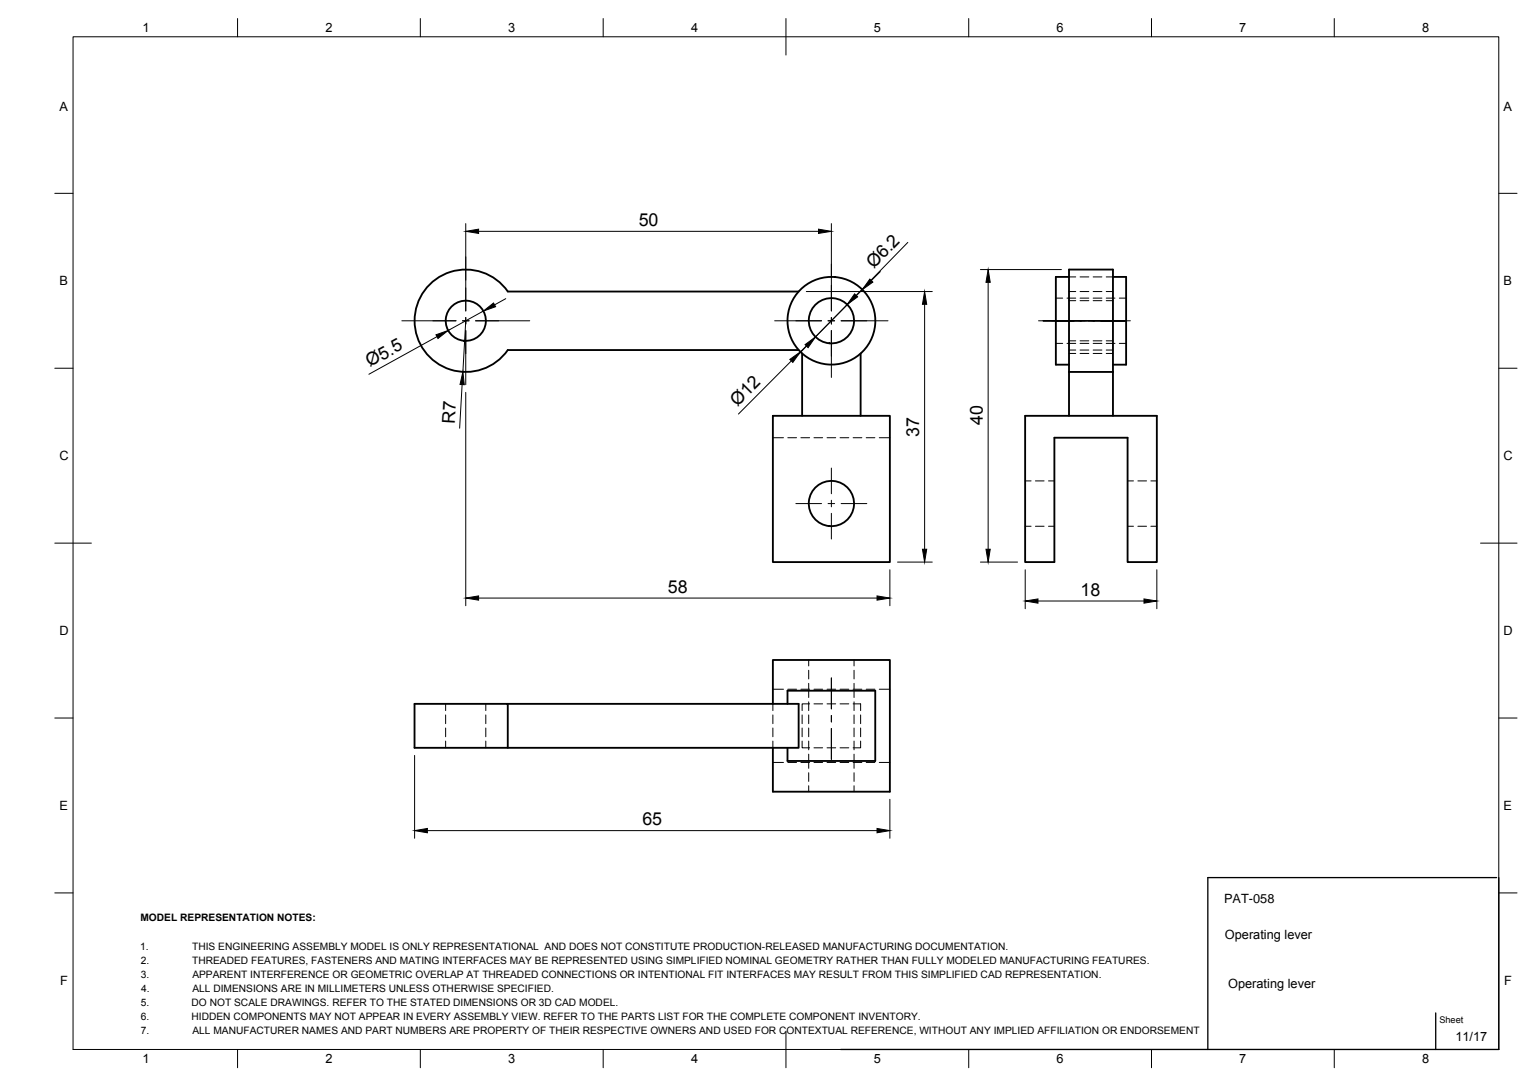
ISO-10303-21;
HEADER;
/* Generated by software containing ST-Developer
 * from STEP Tools, Inc. (www.steptools.com) 
 */

FILE_DESCRIPTION(
/* description */ ('Horizontal push-pull toggle clamp'),
/* implementation_level */ '2;1');

FILE_NAME(
/* name */ 'Operating lever.step',
/* time_stamp */ '2026-10-27T21:21:09-07:00',
/* author */ (''),
/* organization */ (''),
/* preprocessor_version */ 'ST-DEVELOPER v20.2',
/* originating_system */ 'Autodesk Translation Framework v15.17.0.0',
/* authorisation */ '');

FILE_SCHEMA (('AUTOMOTIVE_DESIGN { 1 0 10303 214 3 1 1 }'));
ENDSEC;

DATA;
#10=MECHANICAL_DESIGN_GEOMETRIC_PRESENTATION_REPRESENTATION('',(#186),#4791);
#160=SHAPE_REPRESENTATION_RELATIONSHIP('SRR','None',#4864,#173);
#173=ADVANCED_BREP_SHAPE_REPRESENTATION('',(#199),#4777);
#186=STYLED_ITEM('',(#5009),#199);
#199=MANIFOLD_SOLID_BREP('Body1',#2630);
#223=FACE_BOUND('',#563,.T.);
#224=FACE_BOUND('',#566,.T.);
#225=FACE_BOUND('',#572,.T.);
#226=FACE_BOUND('',#575,.T.);
#227=FACE_BOUND('',#581,.T.);
#228=FACE_BOUND('',#582,.T.);
#229=FACE_BOUND('',#584,.T.);
#230=FACE_BOUND('',#586,.T.);
#231=FACE_BOUND('',#589,.T.);
#232=FACE_BOUND('',#591,.T.);
#233=FACE_BOUND('',#595,.T.);
#283=PLANE('',#2848);
#284=PLANE('',#2850);
#285=PLANE('',#2851);
#286=PLANE('',#2853);
#287=PLANE('',#2860);
#288=PLANE('',#2861);
#289=PLANE('',#2862);
#290=PLANE('',#2863);
#291=PLANE('',#2864);
#292=PLANE('',#2866);
#293=PLANE('',#2867);
#294=PLANE('',#2869);
#295=PLANE('',#2873);
#296=PLANE('',#2874);
#297=PLANE('',#2875);
#298=PLANE('',#2876);
#299=PLANE('',#2877);
#300=PLANE('',#2878);
#301=PLANE('',#2879);
#302=PLANE('',#2880);
#395=FACE_OUTER_BOUND('',#559,.T.);
#396=FACE_OUTER_BOUND('',#560,.T.);
#397=FACE_OUTER_BOUND('',#561,.T.);
#398=FACE_OUTER_BOUND('',#562,.T.);
#399=FACE_OUTER_BOUND('',#564,.T.);
#400=FACE_OUTER_BOUND('',#565,.T.);
#401=FACE_OUTER_BOUND('',#567,.T.);
#402=FACE_OUTER_BOUND('',#568,.T.);
#403=FACE_OUTER_BOUND('',#569,.T.);
#404=FACE_OUTER_BOUND('',#570,.T.);
#405=FACE_OUTER_BOUND('',#571,.T.);
#406=FACE_OUTER_BOUND('',#573,.T.);
#407=FACE_OUTER_BOUND('',#574,.T.);
#408=FACE_OUTER_BOUND('',#576,.T.);
#409=FACE_OUTER_BOUND('',#577,.T.);
#410=FACE_OUTER_BOUND('',#578,.T.);
#411=FACE_OUTER_BOUND('',#579,.T.);
#412=FACE_OUTER_BOUND('',#580,.T.);
#413=FACE_OUTER_BOUND('',#583,.T.);
#414=FACE_OUTER_BOUND('',#585,.T.);
#415=FACE_OUTER_BOUND('',#587,.T.);
#416=FACE_OUTER_BOUND('',#588,.T.);
#417=FACE_OUTER_BOUND('',#590,.T.);
#418=FACE_OUTER_BOUND('',#592,.T.);
#419=FACE_OUTER_BOUND('',#593,.T.);
#420=FACE_OUTER_BOUND('',#594,.T.);
#559=EDGE_LOOP('',(#1951,#1952,#1953,#1954));
#560=EDGE_LOOP('',(#1955,#1956,#1957,#1958));
#561=EDGE_LOOP('',(#1959,#1960,#1961,#1962));
#562=EDGE_LOOP('',(#1963,#1964,#1965,#1966));
#563=EDGE_LOOP('',(#1967));
#564=EDGE_LOOP('',(#1968,#1969,#1970,#1971));
#565=EDGE_LOOP('',(#1972,#1973,#1974,#1975));
#566=EDGE_LOOP('',(#1976));
#567=EDGE_LOOP('',(#1977,#1978,#1979,#1980));
#568=EDGE_LOOP('',(#1981,#1982,#1983,#1984));
#569=EDGE_LOOP('',(#1985,#1986,#1987,#1988));
#570=EDGE_LOOP('',(#1989,#1990,#1991,#1992));
#571=EDGE_LOOP('',(#1993,#1994,#1995,#1996));
#572=EDGE_LOOP('',(#1997));
#573=EDGE_LOOP('',(#1998,#1999,#2000,#2001));
#574=EDGE_LOOP('',(#2002,#2003,#2004,#2005));
#575=EDGE_LOOP('',(#2006));
#576=EDGE_LOOP('',(#2007,#2008,#2009,#2010));
#577=EDGE_LOOP('',(#2011,#2012,#2013,#2014));
#578=EDGE_LOOP('',(#2015,#2016,#2017,#2018));
#579=EDGE_LOOP('',(#2019,#2020,#2021,#2022));
#580=EDGE_LOOP('',(#2023,#2024,#2025,#2026));
#581=EDGE_LOOP('',(#2027,#2028,#2029,#2030));
#582=EDGE_LOOP('',(#2031,#2032,#2033,#2034));
#583=EDGE_LOOP('',(#2035));
#584=EDGE_LOOP('',(#2036));
#585=EDGE_LOOP('',(#2037));
#586=EDGE_LOOP('',(#2038));
#587=EDGE_LOOP('',(#2039,#2040,#2041,#2042,#2043,#2044,#2045,#2046));
#588=EDGE_LOOP('',(#2047,#2048,#2049,#2050));
#589=EDGE_LOOP('',(#2051));
#590=EDGE_LOOP('',(#2052,#2053,#2054,#2055));
#591=EDGE_LOOP('',(#2056,#2057,#2058,#2059));
#592=EDGE_LOOP('',(#2060,#2061,#2062,#2063));
#593=EDGE_LOOP('',(#2064,#2065,#2066,#2067,#2068,#2069,#2070,#2071));
#594=EDGE_LOOP('',(#2072,#2073,#2074,#2075));
#595=EDGE_LOOP('',(#2076));
#724=CIRCLE('',#2840,0.275);
#725=CIRCLE('',#2841,0.275);
#726=CIRCLE('',#2843,0.31);
#727=CIRCLE('',#2844,0.31);
#728=CIRCLE('',#2846,0.7);
#729=CIRCLE('',#2847,0.7);
#730=CIRCLE('',#2849,0.6);
#731=CIRCLE('',#2852,0.6);
#732=CIRCLE('',#2855,0.31);
#733=CIRCLE('',#2856,0.31);
#734=CIRCLE('',#2858,0.31);
#735=CIRCLE('',#2859,0.31);
#736=CIRCLE('',#2865,0.6);
#737=CIRCLE('',#2868,0.6);
#738=CIRCLE('',#2871,0.6);
#739=CIRCLE('',#2872,0.6);
#866=LINE('',#4038,#1086);
#867=LINE('',#4044,#1087);
#868=LINE('',#4049,#1088);
#869=LINE('',#4053,#1089);
#870=LINE('',#4057,#1090);
#871=LINE('',#4060,#1091);
#872=LINE('',#4063,#1092);
#873=LINE('',#4064,#1093);
#874=LINE('',#4067,#1094);
#875=LINE('',#4070,#1095);
#876=LINE('',#4075,#1096);
#877=LINE('',#4081,#1097);
#878=LINE('',#4086,#1098);
#879=LINE('',#4088,#1099);
#880=LINE('',#4090,#1100);
#881=LINE('',#4091,#1101);
#882=LINE('',#4095,#1102);
#883=LINE('',#4097,#1103);
#884=LINE('',#4099,#1104);
#885=LINE('',#4100,#1105);
#886=LINE('',#4104,#1106);
#887=LINE('',#4105,#1107);
#888=LINE('',#4106,#1108);
#889=LINE('',#4108,#1109);
#890=LINE('',#4109,#1110);
#891=LINE('',#4113,#1111);
#892=LINE('',#4115,#1112);
#893=LINE('',#4118,#1113);
#894=LINE('',#4121,#1114);
#895=LINE('',#4123,#1115);
#896=LINE('',#4124,#1116);
#897=LINE('',#4127,#1117);
#898=LINE('',#4129,#1118);
#899=LINE('',#4132,#1119);
#900=LINE('',#4133,#1120);
#901=LINE('',#4138,#1121);
#902=LINE('',#4144,#1122);
#903=LINE('',#4146,#1123);
#904=LINE('',#4148,#1124);
#905=LINE('',#4149,#1125);
#906=LINE('',#4152,#1126);
#907=LINE('',#4153,#1127);
#908=LINE('',#4156,#1128);
#909=LINE('',#4157,#1129);
#910=LINE('',#4160,#1130);
#911=LINE('',#4161,#1131);
#912=LINE('',#4163,#1132);
#1086=VECTOR('',#3248,0.275);
#1087=VECTOR('',#3255,0.31);
#1088=VECTOR('',#3260,1.);
#1089=VECTOR('',#3263,1.);
#1090=VECTOR('',#3268,1.);
#1091=VECTOR('',#3271,1.);
#1092=VECTOR('',#3274,1.);
#1093=VECTOR('',#3275,1.);
#1094=VECTOR('',#3278,1.);
#1095=VECTOR('',#3283,1.);
#1096=VECTOR('',#3288,0.31);
#1097=VECTOR('',#3295,0.31);
#1098=VECTOR('',#3300,1.);
#1099=VECTOR('',#3301,1.);
#1100=VECTOR('',#3302,1.);
#1101=VECTOR('',#3303,1.);
#1102=VECTOR('',#3306,1.);
#1103=VECTOR('',#3307,1.);
#1104=VECTOR('',#3308,1.);
#1105=VECTOR('',#3309,1.);
#1106=VECTOR('',#3312,1.);
#1107=VECTOR('',#3313,1.);
#1108=VECTOR('',#3314,1.);
#1109=VECTOR('',#3317,1.);
#1110=VECTOR('',#3318,1.);
#1111=VECTOR('',#3321,1.);
#1112=VECTOR('',#3322,1.);
#1113=VECTOR('',#3325,1.);
#1114=VECTOR('',#3328,1.);
#1115=VECTOR('',#3329,1.);
#1116=VECTOR('',#3330,1.);
#1117=VECTOR('',#3333,1.);
#1118=VECTOR('',#3334,1.);
#1119=VECTOR('',#3339,1.);
#1120=VECTOR('',#3340,1.);
#1121=VECTOR('',#3345,0.6);
#1122=VECTOR('',#3354,1.);
#1123=VECTOR('',#3355,1.);
#1124=VECTOR('',#3356,1.);
#1125=VECTOR('',#3357,1.);
#1126=VECTOR('',#3360,1.);
#1127=VECTOR('',#3361,1.);
#1128=VECTOR('',#3364,1.);
#1129=VECTOR('',#3365,1.);
#1130=VECTOR('',#3368,1.);
#1131=VECTOR('',#3369,1.);
#1132=VECTOR('',#3372,1.);
#1292=VERTEX_POINT('',#4035);
#1293=VERTEX_POINT('',#4037);
#1294=VERTEX_POINT('',#4041);
#1295=VERTEX_POINT('',#4043);
#1296=VERTEX_POINT('',#4047);
#1297=VERTEX_POINT('',#4048);
#1298=VERTEX_POINT('',#4050);
#1299=VERTEX_POINT('',#4052);
#1300=VERTEX_POINT('',#4056);
#1301=VERTEX_POINT('',#4058);
#1302=VERTEX_POINT('',#4062);
#1303=VERTEX_POINT('',#4066);
#1304=VERTEX_POINT('',#4072);
#1305=VERTEX_POINT('',#4074);
#1306=VERTEX_POINT('',#4078);
#1307=VERTEX_POINT('',#4080);
#1308=VERTEX_POINT('',#4084);
#1309=VERTEX_POINT('',#4085);
#1310=VERTEX_POINT('',#4087);
#1311=VERTEX_POINT('',#4089);
#1312=VERTEX_POINT('',#4093);
#1313=VERTEX_POINT('',#4094);
#1314=VERTEX_POINT('',#4096);
#1315=VERTEX_POINT('',#4098);
#1316=VERTEX_POINT('',#4102);
#1317=VERTEX_POINT('',#4103);
#1318=VERTEX_POINT('',#4111);
#1319=VERTEX_POINT('',#4112);
#1320=VERTEX_POINT('',#4114);
#1321=VERTEX_POINT('',#4116);
#1322=VERTEX_POINT('',#4120);
#1323=VERTEX_POINT('',#4122);
#1324=VERTEX_POINT('',#4126);
#1325=VERTEX_POINT('',#4128);
#1326=VERTEX_POINT('',#4135);
#1327=VERTEX_POINT('',#4137);
#1328=VERTEX_POINT('',#4143);
#1329=VERTEX_POINT('',#4145);
#1330=VERTEX_POINT('',#4147);
#1331=VERTEX_POINT('',#4151);
#1332=VERTEX_POINT('',#4155);
#1333=VERTEX_POINT('',#4159);
#1537=EDGE_CURVE('',#1292,#1292,#724,.T.);
#1538=EDGE_CURVE('',#1292,#1293,#866,.T.);
#1539=EDGE_CURVE('',#1293,#1293,#725,.T.);
#1540=EDGE_CURVE('',#1294,#1294,#726,.T.);
#1541=EDGE_CURVE('',#1294,#1295,#867,.T.);
#1542=EDGE_CURVE('',#1295,#1295,#727,.T.);
#1543=EDGE_CURVE('',#1296,#1297,#868,.T.);
#1544=EDGE_CURVE('',#1298,#1296,#728,.T.);
#1545=EDGE_CURVE('',#1299,#1298,#869,.T.);
#1546=EDGE_CURVE('',#1299,#1297,#729,.T.);
#1547=EDGE_CURVE('',#1300,#1299,#870,.T.);
#1548=EDGE_CURVE('',#1301,#1300,#730,.T.);
#1549=EDGE_CURVE('',#1297,#1301,#871,.T.);
#1550=EDGE_CURVE('',#1302,#1298,#872,.T.);
#1551=EDGE_CURVE('',#1300,#1302,#873,.T.);
#1552=EDGE_CURVE('',#1296,#1303,#874,.T.);
#1553=EDGE_CURVE('',#1302,#1303,#731,.T.);
#1554=EDGE_CURVE('',#1303,#1301,#875,.T.);
#1555=EDGE_CURVE('',#1304,#1304,#732,.T.);
#1556=EDGE_CURVE('',#1304,#1305,#876,.T.);
#1557=EDGE_CURVE('',#1305,#1305,#733,.T.);
#1558=EDGE_CURVE('',#1306,#1306,#734,.T.);
#1559=EDGE_CURVE('',#1306,#1307,#877,.T.);
#1560=EDGE_CURVE('',#1307,#1307,#735,.T.);
#1561=EDGE_CURVE('',#1308,#1309,#878,.T.);
#1562=EDGE_CURVE('',#1308,#1310,#879,.T.);
#1563=EDGE_CURVE('',#1311,#1310,#880,.T.);
#1564=EDGE_CURVE('',#1309,#1311,#881,.T.);
#1565=EDGE_CURVE('',#1312,#1313,#882,.T.);
#1566=EDGE_CURVE('',#1313,#1314,#883,.T.);
#1567=EDGE_CURVE('',#1314,#1315,#884,.T.);
#1568=EDGE_CURVE('',#1315,#1312,#885,.T.);
#1569=EDGE_CURVE('',#1316,#1317,#886,.T.);
#1570=EDGE_CURVE('',#1316,#1314,#887,.T.);
#1571=EDGE_CURVE('',#1317,#1313,#888,.T.);
#1572=EDGE_CURVE('',#1310,#1316,#889,.T.);
#1573=EDGE_CURVE('',#1317,#1311,#890,.T.);
#1574=EDGE_CURVE('',#1318,#1319,#891,.T.);
#1575=EDGE_CURVE('',#1320,#1319,#892,.T.);
#1576=EDGE_CURVE('',#1321,#1320,#736,.T.);
#1577=EDGE_CURVE('',#1318,#1321,#893,.T.);
#1578=EDGE_CURVE('',#1319,#1322,#894,.T.);
#1579=EDGE_CURVE('',#1323,#1322,#895,.T.);
#1580=EDGE_CURVE('',#1320,#1323,#896,.T.);
#1581=EDGE_CURVE('',#1322,#1324,#897,.T.);
#1582=EDGE_CURVE('',#1324,#1325,#898,.T.);
#1583=EDGE_CURVE('',#1323,#1325,#737,.T.);
#1584=EDGE_CURVE('',#1324,#1318,#899,.T.);
#1585=EDGE_CURVE('',#1325,#1321,#900,.T.);
#1586=EDGE_CURVE('',#1326,#1326,#738,.T.);
#1587=EDGE_CURVE('',#1326,#1327,#901,.T.);
#1588=EDGE_CURVE('',#1327,#1327,#739,.T.);
#1589=EDGE_CURVE('',#1328,#1308,#902,.T.);
#1590=EDGE_CURVE('',#1329,#1328,#903,.T.);
#1591=EDGE_CURVE('',#1330,#1329,#904,.T.);
#1592=EDGE_CURVE('',#1330,#1315,#905,.T.);
#1593=EDGE_CURVE('',#1309,#1331,#906,.T.);
#1594=EDGE_CURVE('',#1331,#1328,#907,.T.);
#1595=EDGE_CURVE('',#1332,#1330,#908,.T.);
#1596=EDGE_CURVE('',#1332,#1312,#909,.T.);
#1597=EDGE_CURVE('',#1329,#1333,#910,.T.);
#1598=EDGE_CURVE('',#1333,#1331,#911,.T.);
#1599=EDGE_CURVE('',#1333,#1332,#912,.T.);
#1951=ORIENTED_EDGE('',*,*,#1537,.F.);
#1952=ORIENTED_EDGE('',*,*,#1538,.T.);
#1953=ORIENTED_EDGE('',*,*,#1539,.F.);
#1954=ORIENTED_EDGE('',*,*,#1538,.F.);
#1955=ORIENTED_EDGE('',*,*,#1540,.F.);
#1956=ORIENTED_EDGE('',*,*,#1541,.T.);
#1957=ORIENTED_EDGE('',*,*,#1542,.F.);
#1958=ORIENTED_EDGE('',*,*,#1541,.F.);
#1959=ORIENTED_EDGE('',*,*,#1543,.F.);
#1960=ORIENTED_EDGE('',*,*,#1544,.F.);
#1961=ORIENTED_EDGE('',*,*,#1545,.F.);
#1962=ORIENTED_EDGE('',*,*,#1546,.T.);
#1963=ORIENTED_EDGE('',*,*,#1546,.F.);
#1964=ORIENTED_EDGE('',*,*,#1547,.F.);
#1965=ORIENTED_EDGE('',*,*,#1548,.F.);
#1966=ORIENTED_EDGE('',*,*,#1549,.F.);
#1967=ORIENTED_EDGE('',*,*,#1537,.T.);
#1968=ORIENTED_EDGE('',*,*,#1545,.T.);
#1969=ORIENTED_EDGE('',*,*,#1550,.F.);
#1970=ORIENTED_EDGE('',*,*,#1551,.F.);
#1971=ORIENTED_EDGE('',*,*,#1547,.T.);
#1972=ORIENTED_EDGE('',*,*,#1552,.T.);
#1973=ORIENTED_EDGE('',*,*,#1553,.F.);
#1974=ORIENTED_EDGE('',*,*,#1550,.T.);
#1975=ORIENTED_EDGE('',*,*,#1544,.T.);
#1976=ORIENTED_EDGE('',*,*,#1539,.T.);
#1977=ORIENTED_EDGE('',*,*,#1543,.T.);
#1978=ORIENTED_EDGE('',*,*,#1549,.T.);
#1979=ORIENTED_EDGE('',*,*,#1554,.F.);
#1980=ORIENTED_EDGE('',*,*,#1552,.F.);
#1981=ORIENTED_EDGE('',*,*,#1555,.F.);
#1982=ORIENTED_EDGE('',*,*,#1556,.T.);
#1983=ORIENTED_EDGE('',*,*,#1557,.F.);
#1984=ORIENTED_EDGE('',*,*,#1556,.F.);
#1985=ORIENTED_EDGE('',*,*,#1558,.F.);
#1986=ORIENTED_EDGE('',*,*,#1559,.T.);
#1987=ORIENTED_EDGE('',*,*,#1560,.F.);
#1988=ORIENTED_EDGE('',*,*,#1559,.F.);
#1989=ORIENTED_EDGE('',*,*,#1561,.F.);
#1990=ORIENTED_EDGE('',*,*,#1562,.T.);
#1991=ORIENTED_EDGE('',*,*,#1563,.F.);
#1992=ORIENTED_EDGE('',*,*,#1564,.F.);
#1993=ORIENTED_EDGE('',*,*,#1565,.T.);
#1994=ORIENTED_EDGE('',*,*,#1566,.T.);
#1995=ORIENTED_EDGE('',*,*,#1567,.T.);
#1996=ORIENTED_EDGE('',*,*,#1568,.T.);
#1997=ORIENTED_EDGE('',*,*,#1560,.T.);
#1998=ORIENTED_EDGE('',*,*,#1569,.F.);
#1999=ORIENTED_EDGE('',*,*,#1570,.T.);
#2000=ORIENTED_EDGE('',*,*,#1566,.F.);
#2001=ORIENTED_EDGE('',*,*,#1571,.F.);
#2002=ORIENTED_EDGE('',*,*,#1563,.T.);
#2003=ORIENTED_EDGE('',*,*,#1572,.T.);
#2004=ORIENTED_EDGE('',*,*,#1569,.T.);
#2005=ORIENTED_EDGE('',*,*,#1573,.T.);
#2006=ORIENTED_EDGE('',*,*,#1558,.T.);
#2007=ORIENTED_EDGE('',*,*,#1574,.T.);
#2008=ORIENTED_EDGE('',*,*,#1575,.F.);
#2009=ORIENTED_EDGE('',*,*,#1576,.F.);
#2010=ORIENTED_EDGE('',*,*,#1577,.F.);
#2011=ORIENTED_EDGE('',*,*,#1578,.T.);
#2012=ORIENTED_EDGE('',*,*,#1579,.F.);
#2013=ORIENTED_EDGE('',*,*,#1580,.F.);
#2014=ORIENTED_EDGE('',*,*,#1575,.T.);
#2015=ORIENTED_EDGE('',*,*,#1581,.T.);
#2016=ORIENTED_EDGE('',*,*,#1582,.T.);
#2017=ORIENTED_EDGE('',*,*,#1583,.F.);
#2018=ORIENTED_EDGE('',*,*,#1579,.T.);
#2019=ORIENTED_EDGE('',*,*,#1584,.T.);
#2020=ORIENTED_EDGE('',*,*,#1577,.T.);
#2021=ORIENTED_EDGE('',*,*,#1585,.F.);
#2022=ORIENTED_EDGE('',*,*,#1582,.F.);
#2023=ORIENTED_EDGE('',*,*,#1586,.F.);
#2024=ORIENTED_EDGE('',*,*,#1587,.T.);
#2025=ORIENTED_EDGE('',*,*,#1588,.T.);
#2026=ORIENTED_EDGE('',*,*,#1587,.F.);
#2027=ORIENTED_EDGE('',*,*,#1551,.T.);
#2028=ORIENTED_EDGE('',*,*,#1553,.T.);
#2029=ORIENTED_EDGE('',*,*,#1554,.T.);
#2030=ORIENTED_EDGE('',*,*,#1548,.T.);
#2031=ORIENTED_EDGE('',*,*,#1580,.T.);
#2032=ORIENTED_EDGE('',*,*,#1583,.T.);
#2033=ORIENTED_EDGE('',*,*,#1585,.T.);
#2034=ORIENTED_EDGE('',*,*,#1576,.T.);
#2035=ORIENTED_EDGE('',*,*,#1586,.T.);
#2036=ORIENTED_EDGE('',*,*,#1542,.T.);
#2037=ORIENTED_EDGE('',*,*,#1588,.F.);
#2038=ORIENTED_EDGE('',*,*,#1540,.T.);
#2039=ORIENTED_EDGE('',*,*,#1589,.F.);
#2040=ORIENTED_EDGE('',*,*,#1590,.F.);
#2041=ORIENTED_EDGE('',*,*,#1591,.F.);
#2042=ORIENTED_EDGE('',*,*,#1592,.T.);
#2043=ORIENTED_EDGE('',*,*,#1567,.F.);
#2044=ORIENTED_EDGE('',*,*,#1570,.F.);
#2045=ORIENTED_EDGE('',*,*,#1572,.F.);
#2046=ORIENTED_EDGE('',*,*,#1562,.F.);
#2047=ORIENTED_EDGE('',*,*,#1561,.T.);
#2048=ORIENTED_EDGE('',*,*,#1593,.T.);
#2049=ORIENTED_EDGE('',*,*,#1594,.T.);
#2050=ORIENTED_EDGE('',*,*,#1589,.T.);
#2051=ORIENTED_EDGE('',*,*,#1557,.T.);
#2052=ORIENTED_EDGE('',*,*,#1595,.F.);
#2053=ORIENTED_EDGE('',*,*,#1596,.T.);
#2054=ORIENTED_EDGE('',*,*,#1568,.F.);
#2055=ORIENTED_EDGE('',*,*,#1592,.F.);
#2056=ORIENTED_EDGE('',*,*,#1581,.F.);
#2057=ORIENTED_EDGE('',*,*,#1578,.F.);
#2058=ORIENTED_EDGE('',*,*,#1574,.F.);
#2059=ORIENTED_EDGE('',*,*,#1584,.F.);
#2060=ORIENTED_EDGE('',*,*,#1597,.F.);
#2061=ORIENTED_EDGE('',*,*,#1590,.T.);
#2062=ORIENTED_EDGE('',*,*,#1594,.F.);
#2063=ORIENTED_EDGE('',*,*,#1598,.F.);
#2064=ORIENTED_EDGE('',*,*,#1599,.F.);
#2065=ORIENTED_EDGE('',*,*,#1598,.T.);
#2066=ORIENTED_EDGE('',*,*,#1593,.F.);
#2067=ORIENTED_EDGE('',*,*,#1564,.T.);
#2068=ORIENTED_EDGE('',*,*,#1573,.F.);
#2069=ORIENTED_EDGE('',*,*,#1571,.T.);
#2070=ORIENTED_EDGE('',*,*,#1565,.F.);
#2071=ORIENTED_EDGE('',*,*,#1596,.F.);
#2072=ORIENTED_EDGE('',*,*,#1591,.T.);
#2073=ORIENTED_EDGE('',*,*,#1597,.T.);
#2074=ORIENTED_EDGE('',*,*,#1599,.T.);
#2075=ORIENTED_EDGE('',*,*,#1595,.T.);
#2076=ORIENTED_EDGE('',*,*,#1555,.T.);
#2449=CYLINDRICAL_SURFACE('',#2839,0.275);
#2450=CYLINDRICAL_SURFACE('',#2842,0.31);
#2451=CYLINDRICAL_SURFACE('',#2845,0.7);
#2452=CYLINDRICAL_SURFACE('',#2854,0.31);
#2453=CYLINDRICAL_SURFACE('',#2857,0.31);
#2454=CYLINDRICAL_SURFACE('',#2870,0.6);
#2511=ADVANCED_FACE('',(#395),#2449,.F.);
#2512=ADVANCED_FACE('',(#396),#2450,.F.);
#2513=ADVANCED_FACE('',(#397),#2451,.T.);
#2514=ADVANCED_FACE('',(#398,#223),#283,.F.);
#2515=ADVANCED_FACE('',(#399),#284,.T.);
#2516=ADVANCED_FACE('',(#400,#224),#285,.T.);
#2517=ADVANCED_FACE('',(#401),#286,.T.);
#2518=ADVANCED_FACE('',(#402),#2452,.F.);
#2519=ADVANCED_FACE('',(#403),#2453,.F.);
#2520=ADVANCED_FACE('',(#404),#287,.T.);
#2521=ADVANCED_FACE('',(#405,#225),#288,.T.);
#2522=ADVANCED_FACE('',(#406),#289,.T.);
#2523=ADVANCED_FACE('',(#407,#226),#290,.F.);
#2524=ADVANCED_FACE('',(#408),#291,.F.);
#2525=ADVANCED_FACE('',(#409),#292,.T.);
#2526=ADVANCED_FACE('',(#410),#293,.T.);
#2527=ADVANCED_FACE('',(#411),#294,.T.);
#2528=ADVANCED_FACE('',(#412,#227,#228),#2454,.T.);
#2529=ADVANCED_FACE('',(#413,#229),#295,.T.);
#2530=ADVANCED_FACE('',(#414,#230),#296,.F.);
#2531=ADVANCED_FACE('',(#415),#297,.T.);
#2532=ADVANCED_FACE('',(#416,#231),#298,.T.);
#2533=ADVANCED_FACE('',(#417,#232),#299,.T.);
#2534=ADVANCED_FACE('',(#418),#300,.T.);
#2535=ADVANCED_FACE('',(#419),#301,.T.);
#2536=ADVANCED_FACE('',(#420,#233),#302,.F.);
#2630=CLOSED_SHELL('',(#2511,#2512,#2513,#2514,#2515,#2516,#2517,#2518,
#2519,#2520,#2521,#2522,#2523,#2524,#2525,#2526,#2527,#2528,#2529,#2530,
#2531,#2532,#2533,#2534,#2535,#2536));
#2838=AXIS2_PLACEMENT_3D('',#4033,#3242,#3243);
#2839=AXIS2_PLACEMENT_3D('',#4034,#3244,#3245);
#2840=AXIS2_PLACEMENT_3D('',#4036,#3246,#3247);
#2841=AXIS2_PLACEMENT_3D('',#4039,#3249,#3250);
#2842=AXIS2_PLACEMENT_3D('',#4040,#3251,#3252);
#2843=AXIS2_PLACEMENT_3D('',#4042,#3253,#3254);
#2844=AXIS2_PLACEMENT_3D('',#4045,#3256,#3257);
#2845=AXIS2_PLACEMENT_3D('',#4046,#3258,#3259);
#2846=AXIS2_PLACEMENT_3D('',#4051,#3261,#3262);
#2847=AXIS2_PLACEMENT_3D('',#4054,#3264,#3265);
#2848=AXIS2_PLACEMENT_3D('',#4055,#3266,#3267);
#2849=AXIS2_PLACEMENT_3D('',#4059,#3269,#3270);
#2850=AXIS2_PLACEMENT_3D('',#4061,#3272,#3273);
#2851=AXIS2_PLACEMENT_3D('',#4065,#3276,#3277);
#2852=AXIS2_PLACEMENT_3D('',#4068,#3279,#3280);
#2853=AXIS2_PLACEMENT_3D('',#4069,#3281,#3282);
#2854=AXIS2_PLACEMENT_3D('',#4071,#3284,#3285);
#2855=AXIS2_PLACEMENT_3D('',#4073,#3286,#3287);
#2856=AXIS2_PLACEMENT_3D('',#4076,#3289,#3290);
#2857=AXIS2_PLACEMENT_3D('',#4077,#3291,#3292);
#2858=AXIS2_PLACEMENT_3D('',#4079,#3293,#3294);
#2859=AXIS2_PLACEMENT_3D('',#4082,#3296,#3297);
#2860=AXIS2_PLACEMENT_3D('',#4083,#3298,#3299);
#2861=AXIS2_PLACEMENT_3D('',#4092,#3304,#3305);
#2862=AXIS2_PLACEMENT_3D('',#4101,#3310,#3311);
#2863=AXIS2_PLACEMENT_3D('',#4107,#3315,#3316);
#2864=AXIS2_PLACEMENT_3D('',#4110,#3319,#3320);
#2865=AXIS2_PLACEMENT_3D('',#4117,#3323,#3324);
#2866=AXIS2_PLACEMENT_3D('',#4119,#3326,#3327);
#2867=AXIS2_PLACEMENT_3D('',#4125,#3331,#3332);
#2868=AXIS2_PLACEMENT_3D('',#4130,#3335,#3336);
#2869=AXIS2_PLACEMENT_3D('',#4131,#3337,#3338);
#2870=AXIS2_PLACEMENT_3D('',#4134,#3341,#3342);
#2871=AXIS2_PLACEMENT_3D('',#4136,#3343,#3344);
#2872=AXIS2_PLACEMENT_3D('',#4139,#3346,#3347);
#2873=AXIS2_PLACEMENT_3D('',#4140,#3348,#3349);
#2874=AXIS2_PLACEMENT_3D('',#4141,#3350,#3351);
#2875=AXIS2_PLACEMENT_3D('',#4142,#3352,#3353);
#2876=AXIS2_PLACEMENT_3D('',#4150,#3358,#3359);
#2877=AXIS2_PLACEMENT_3D('',#4154,#3362,#3363);
#2878=AXIS2_PLACEMENT_3D('',#4158,#3366,#3367);
#2879=AXIS2_PLACEMENT_3D('',#4162,#3370,#3371);
#2880=AXIS2_PLACEMENT_3D('',#4164,#3373,#3374);
#3242=DIRECTION('axis',(0.,0.,1.));
#3243=DIRECTION('refdir',(1.,0.,0.));
#3244=DIRECTION('center_axis',(0.,1.,0.));
#3245=DIRECTION('ref_axis',(1.,0.,0.));
#3246=DIRECTION('center_axis',(0.,1.,0.));
#3247=DIRECTION('ref_axis',(1.,0.,0.));
#3248=DIRECTION('',(0.,1.,0.));
#3249=DIRECTION('center_axis',(0.,-1.,0.));
#3250=DIRECTION('ref_axis',(1.,0.,0.));
#3251=DIRECTION('center_axis',(0.,1.,0.));
#3252=DIRECTION('ref_axis',(1.,0.,0.));
#3253=DIRECTION('center_axis',(0.,1.,0.));
#3254=DIRECTION('ref_axis',(1.,0.,0.));
#3255=DIRECTION('',(0.,1.,0.));
#3256=DIRECTION('center_axis',(0.,-1.,0.));
#3257=DIRECTION('ref_axis',(1.,0.,0.));
#3258=DIRECTION('center_axis',(0.,1.,0.));
#3259=DIRECTION('ref_axis',(0.0871557427476581,0.,0.996194698091746));
#3260=DIRECTION('',(0.,-1.,0.));
#3261=DIRECTION('center_axis',(0.,1.,0.));
#3262=DIRECTION('ref_axis',(1.,0.,0.));
#3263=DIRECTION('',(0.,1.,0.));
#3264=DIRECTION('center_axis',(0.,1.,0.));
#3265=DIRECTION('ref_axis',(1.,0.,0.));
#3266=DIRECTION('center_axis',(0.,1.,0.));
#3267=DIRECTION('ref_axis',(1.,0.,0.));
#3268=DIRECTION('',(0.0871557427476582,0.,0.996194698091746));
#3269=DIRECTION('center_axis',(0.,-1.,0.));
#3270=DIRECTION('ref_axis',(1.,0.,0.));
#3271=DIRECTION('',(-0.0871557427476581,0.,-0.996194698091746));
#3272=DIRECTION('center_axis',(-0.996194698091746,0.,0.0871557427476582));
#3273=DIRECTION('ref_axis',(0.0871557427476582,0.,0.996194698091746));
#3274=DIRECTION('',(0.0871557427476582,0.,0.996194698091746));
#3275=DIRECTION('',(0.,1.,0.));
#3276=DIRECTION('center_axis',(0.,1.,0.));
#3277=DIRECTION('ref_axis',(0.,0.,1.));
#3278=DIRECTION('',(-0.0871557427476581,0.,-0.996194698091746));
#3279=DIRECTION('center_axis',(0.,1.,0.));
#3280=DIRECTION('ref_axis',(1.,0.,0.));
#3281=DIRECTION('center_axis',(0.996194698091746,0.,-0.0871557427476581));
#3282=DIRECTION('ref_axis',(-0.0871557427476581,0.,-0.996194698091746));
#3283=DIRECTION('',(0.,-1.,0.));
#3284=DIRECTION('center_axis',(0.,1.,0.));
#3285=DIRECTION('ref_axis',(1.,0.,0.));
#3286=DIRECTION('center_axis',(0.,1.,0.));
#3287=DIRECTION('ref_axis',(1.,0.,0.));
#3288=DIRECTION('',(0.,1.,0.));
#3289=DIRECTION('center_axis',(0.,-1.,0.));
#3290=DIRECTION('ref_axis',(1.,0.,0.));
#3291=DIRECTION('center_axis',(0.,1.,0.));
#3292=DIRECTION('ref_axis',(1.,0.,0.));
#3293=DIRECTION('center_axis',(0.,1.,0.));
#3294=DIRECTION('ref_axis',(1.,0.,0.));
#3295=DIRECTION('',(0.,1.,0.));
#3296=DIRECTION('center_axis',(0.,-1.,0.));
#3297=DIRECTION('ref_axis',(1.,0.,0.));
#3298=DIRECTION('center_axis',(0.996194698091746,0.,-0.0871557427476583));
#3299=DIRECTION('ref_axis',(-0.0871557427476583,0.,-0.996194698091746));
#3300=DIRECTION('',(0.0871557427476583,0.,0.996194698091746));
#3301=DIRECTION('',(0.,1.,0.));
#3302=DIRECTION('',(-0.0871557427476583,0.,-0.996194698091746));
#3303=DIRECTION('',(0.,1.,0.));
#3304=DIRECTION('center_axis',(0.,1.,0.));
#3305=DIRECTION('ref_axis',(0.,0.,1.));
#3306=DIRECTION('',(0.996194698091746,0.,-0.0871557427476581));
#3307=DIRECTION('',(-0.087155742747658,0.,-0.996194698091746));
#3308=DIRECTION('',(-0.996194698091746,0.,0.0871557427476581));
#3309=DIRECTION('',(0.0871557427476582,0.,0.996194698091746));
#3310=DIRECTION('center_axis',(0.996194698091746,0.,-0.087155742747658));
#3311=DIRECTION('ref_axis',(-0.087155742747658,0.,-0.996194698091746));
#3312=DIRECTION('',(0.087155742747658,0.,0.996194698091746));
#3313=DIRECTION('',(0.,1.,0.));
#3314=DIRECTION('',(0.,1.,0.));
#3315=DIRECTION('center_axis',(0.,1.,0.));
#3316=DIRECTION('ref_axis',(1.,0.,0.));
#3317=DIRECTION('',(0.996194698091746,0.,-0.0871557427476581));
#3318=DIRECTION('',(-0.996194698091746,0.,0.0871557427476581));
#3319=DIRECTION('center_axis',(0.,1.,0.));
#3320=DIRECTION('ref_axis',(1.,0.,0.));
#3321=DIRECTION('',(0.0871557427476582,0.,0.996194698091746));
#3322=DIRECTION('',(0.996194698091746,0.,-0.0871557427476581));
#3323=DIRECTION('center_axis',(0.,-1.,0.));
#3324=DIRECTION('ref_axis',(1.,0.,0.));
#3325=DIRECTION('',(-0.996194698091746,0.,0.087155742747658));
#3326=DIRECTION('center_axis',(0.0871557427476581,0.,0.996194698091746));
#3327=DIRECTION('ref_axis',(0.996194698091746,0.,-0.0871557427476581));
#3328=DIRECTION('',(0.,1.,0.));
#3329=DIRECTION('',(0.996194698091746,0.,-0.0871557427476581));
#3330=DIRECTION('',(0.,1.,0.));
#3331=DIRECTION('center_axis',(0.,1.,0.));
#3332=DIRECTION('ref_axis',(0.,0.,1.));
#3333=DIRECTION('',(-0.0871557427476582,0.,-0.996194698091746));
#3334=DIRECTION('',(-0.996194698091746,0.,0.087155742747658));
#3335=DIRECTION('center_axis',(0.,1.,0.));
#3336=DIRECTION('ref_axis',(1.,0.,0.));
#3337=DIRECTION('center_axis',(-0.087155742747658,0.,-0.996194698091746));
#3338=DIRECTION('ref_axis',(-0.996194698091746,0.,0.087155742747658));
#3339=DIRECTION('',(0.,-1.,0.));
#3340=DIRECTION('',(0.,-1.,0.));
#3341=DIRECTION('center_axis',(0.,1.,0.));
#3342=DIRECTION('ref_axis',(1.,0.,0.));
#3343=DIRECTION('center_axis',(0.,1.,0.));
#3344=DIRECTION('ref_axis',(1.,0.,0.));
#3345=DIRECTION('',(0.,-1.,0.));
#3346=DIRECTION('center_axis',(0.,1.,0.));
#3347=DIRECTION('ref_axis',(1.,0.,0.));
#3348=DIRECTION('center_axis',(0.,1.,0.));
#3349=DIRECTION('ref_axis',(1.,0.,0.));
#3350=DIRECTION('center_axis',(0.,1.,0.));
#3351=DIRECTION('ref_axis',(1.,0.,0.));
#3352=DIRECTION('center_axis',(-0.0871557427476581,0.,-0.996194698091746));
#3353=DIRECTION('ref_axis',(-0.996194698091746,0.,0.0871557427476581));
#3354=DIRECTION('',(-0.996194698091746,0.,0.0871557427476581));
#3355=DIRECTION('',(0.,1.,0.));
#3356=DIRECTION('',(0.996194698091746,0.,-0.0871557427476581));
#3357=DIRECTION('',(0.,1.,0.));
#3358=DIRECTION('center_axis',(0.,1.,0.));
#3359=DIRECTION('ref_axis',(0.,0.,1.));
#3360=DIRECTION('',(0.996194698091746,0.,-0.0871557427476581));
#3361=DIRECTION('',(-0.087155742747658,0.,-0.996194698091746));
#3362=DIRECTION('center_axis',(-0.996194698091746,0.,0.0871557427476582));
#3363=DIRECTION('ref_axis',(0.0871557427476582,0.,0.996194698091746));
#3364=DIRECTION('',(-0.0871557427476582,0.,-0.996194698091746));
#3365=DIRECTION('',(0.,1.,0.));
#3366=DIRECTION('center_axis',(0.996194698091746,0.,-0.087155742747658));
#3367=DIRECTION('ref_axis',(-0.087155742747658,0.,-0.996194698091746));
#3368=DIRECTION('',(0.087155742747658,0.,0.996194698091746));
#3369=DIRECTION('',(0.,1.,0.));
#3370=DIRECTION('center_axis',(0.0871557427476581,0.,0.996194698091746));
#3371=DIRECTION('ref_axis',(0.996194698091746,0.,-0.0871557427476581));
#3372=DIRECTION('',(-0.996194698091746,0.,0.0871557427476581));
#3373=DIRECTION('center_axis',(0.,1.,0.));
#3374=DIRECTION('ref_axis',(1.,0.,0.));
#4033=CARTESIAN_POINT('',(0.,0.,0.));
#4034=CARTESIAN_POINT('Origin',(0.435778713738291,-0.4,7.48097349045873));
#4035=CARTESIAN_POINT('',(0.160778713738291,-0.3,7.48097349045873));
#4036=CARTESIAN_POINT('Origin',(0.435778713738291,-0.3,7.48097349045873));
#4037=CARTESIAN_POINT('',(0.160778713738291,0.3,7.48097349045873));
#4038=CARTESIAN_POINT('',(0.160778713738291,-0.4,7.48097349045873));
#4039=CARTESIAN_POINT('Origin',(0.435778713738291,0.3,7.48097349045873));
#4040=CARTESIAN_POINT('Origin',(0.,-0.6,2.5));
#4041=CARTESIAN_POINT('',(-0.31,-0.48,2.5));
#4042=CARTESIAN_POINT('Origin',(0.,-0.48,2.5));
#4043=CARTESIAN_POINT('',(-0.31,0.48,2.5));
#4044=CARTESIAN_POINT('',(-0.31,-0.6,2.5));
#4045=CARTESIAN_POINT('Origin',(0.,0.48,2.5));
#4046=CARTESIAN_POINT('Origin',(0.435778713738291,-0.3,7.48097349045873));
#4047=CARTESIAN_POINT('',(0.784189430553042,0.3,6.87384090822596));
#4048=CARTESIAN_POINT('',(0.784189430553042,-0.3,6.87384090822596));
#4049=CARTESIAN_POINT('',(0.784189430553042,-0.3,6.87384090822596));
#4050=CARTESIAN_POINT('',(-0.0127663279203548,0.3,6.94356550242408));
#4051=CARTESIAN_POINT('Origin',(0.435778713738291,0.3,7.48097349045873));
#4052=CARTESIAN_POINT('',(-0.0127663279203548,-0.3,6.94356550242408));
#4053=CARTESIAN_POINT('',(-0.0127663279203548,-0.3,6.94356550242408));
#4054=CARTESIAN_POINT('Origin',(0.435778713738291,-0.3,7.48097349045873));
#4055=CARTESIAN_POINT('Origin',(0.217889356869145,-0.3,4.99048674522937));
#4056=CARTESIAN_POINT('',(-0.359500646154049,-0.3,2.98037410985067));
#4057=CARTESIAN_POINT('',(-0.398477879236698,-0.3,2.53486229709906));
#4058=CARTESIAN_POINT('',(0.437455112319348,-0.3,2.91064951565254));
#4059=CARTESIAN_POINT('Origin',(0.,-0.3,2.5));
#4060=CARTESIAN_POINT('',(0.834256592974989,-0.3,7.44611119335967));
#4061=CARTESIAN_POINT('Origin',(-0.398477879236698,-0.3,2.53486229709906));
#4062=CARTESIAN_POINT('',(-0.359500646154049,0.3,2.98037410985067));
#4063=CARTESIAN_POINT('',(-0.398477879236698,0.3,2.53486229709906));
#4064=CARTESIAN_POINT('',(-0.359500646154049,-0.48,2.98037410985067));
#4065=CARTESIAN_POINT('Origin',(0.217889356869145,0.3,4.99048674522937));
#4066=CARTESIAN_POINT('',(0.437455112319348,0.3,2.91064951565254));
#4067=CARTESIAN_POINT('',(0.834256592974989,0.3,7.44611119335967));
#4068=CARTESIAN_POINT('Origin',(0.,0.3,2.5));
#4069=CARTESIAN_POINT('Origin',(0.834256592974989,-0.3,7.44611119335967));
#4070=CARTESIAN_POINT('',(0.437455112319348,-0.48,2.91064951565254));
#4071=CARTESIAN_POINT('Origin',(2.49048674522936,-1.,2.28211064313085));
#4072=CARTESIAN_POINT('',(2.18048674522936,-0.9,2.28211064313085));
#4073=CARTESIAN_POINT('Origin',(2.49048674522936,-0.9,2.28211064313085));
#4074=CARTESIAN_POINT('',(2.18048674522936,-0.5,2.28211064313085));
#4075=CARTESIAN_POINT('',(2.18048674522936,-1.,2.28211064313085));
#4076=CARTESIAN_POINT('Origin',(2.49048674522936,-0.5,2.28211064313085));
#4077=CARTESIAN_POINT('Origin',(2.49048674522936,-1.,2.28211064313085));
#4078=CARTESIAN_POINT('',(2.18048674522936,0.5,2.28211064313085));
#4079=CARTESIAN_POINT('Origin',(2.49048674522936,0.5,2.28211064313085));
#4080=CARTESIAN_POINT('',(2.18048674522936,0.9,2.28211064313085));
#4081=CARTESIAN_POINT('',(2.18048674522936,-1.,2.28211064313085));
#4082=CARTESIAN_POINT('Origin',(2.49048674522936,0.9,2.28211064313085));
#4083=CARTESIAN_POINT('Origin',(1.66363611114492,-0.9,3.15750657007714));
#4084=CARTESIAN_POINT('',(1.52418692274867,-0.5,1.56359505313035));
#4085=CARTESIAN_POINT('',(1.66363611114492,-0.5,3.15750657007714));
#4086=CARTESIAN_POINT('',(1.62877381404586,-0.5,2.75902869084045));
#4087=CARTESIAN_POINT('',(1.52418692274867,0.5,1.56359505313035));
#4088=CARTESIAN_POINT('',(1.52418692274867,-0.9,1.56359505313035));
#4089=CARTESIAN_POINT('',(1.66363611114492,0.5,3.15750657007714));
#4090=CARTESIAN_POINT('',(1.62877381404586,0.5,2.75902869084045));
#4091=CARTESIAN_POINT('',(1.66363611114492,-0.9,3.15750657007714));
#4092=CARTESIAN_POINT('Origin',(2.29124780561101,0.9,2.29954179168039));
#4093=CARTESIAN_POINT('',(1.3647777017174,0.9,3.18365329290144));
#4094=CARTESIAN_POINT('',(3.35716709790089,0.9,3.00934180740612));
#4095=CARTESIAN_POINT('',(3.35716709790089,0.9,3.00934180740612));
#4096=CARTESIAN_POINT('',(3.21771790950463,0.9,1.41543029045933));
#4097=CARTESIAN_POINT('',(3.21771790950463,0.9,1.41543029045933));
#4098=CARTESIAN_POINT('',(1.22532851332114,0.9,1.58974177595465));
#4099=CARTESIAN_POINT('',(1.22532851332114,0.9,1.58974177595465));
#4100=CARTESIAN_POINT('',(1.3647777017174,0.9,3.18365329290144));
#4101=CARTESIAN_POINT('Origin',(3.35716709790089,0.5,3.00934180740612));
#4102=CARTESIAN_POINT('',(3.21771790950463,0.5,1.41543029045933));
#4103=CARTESIAN_POINT('',(3.35716709790089,0.5,3.00934180740612));
#4104=CARTESIAN_POINT('',(3.21771790950463,0.5,1.41543029045933));
#4105=CARTESIAN_POINT('',(3.21771790950463,0.5,1.41543029045933));
#4106=CARTESIAN_POINT('',(3.35716709790089,0.5,3.00934180740612));
#4107=CARTESIAN_POINT('Origin',(2.29124780561101,0.5,2.29954179168039));
#4108=CARTESIAN_POINT('',(1.22532851332114,0.5,1.58974177595465));
#4109=CARTESIAN_POINT('',(3.35716709790089,0.5,3.00934180740612));
#4110=CARTESIAN_POINT('Origin',(0.747146023568809,-0.3,2.43463319293926));
#4111=CARTESIAN_POINT('',(1.26019081042021,-0.3,1.98821965519135));
#4112=CARTESIAN_POINT('',(1.32991540461833,-0.3,2.78517541366474));
#4113=CARTESIAN_POINT('',(1.26019081042021,-0.3,1.98821965519135));
#4114=CARTESIAN_POINT('',(0.480374109850668,-0.3,2.85950064615405));
#4115=CARTESIAN_POINT('',(0.0348622970990633,-0.3,2.8984778792367));
#4116=CARTESIAN_POINT('',(0.410649515652541,-0.3,2.06254488768065));
#4117=CARTESIAN_POINT('Origin',(0.,-0.3,2.5));
#4118=CARTESIAN_POINT('',(1.45942975003856,-0.3,1.97078850664181));
#4119=CARTESIAN_POINT('Origin',(0.0348622970990633,-0.3,2.8984778792367));
#4120=CARTESIAN_POINT('',(1.32991540461833,0.3,2.78517541366474));
#4121=CARTESIAN_POINT('',(1.32991540461833,-0.6,2.78517541366474));
#4122=CARTESIAN_POINT('',(0.480374109850668,0.3,2.85950064615405));
#4123=CARTESIAN_POINT('',(0.0348622970990633,0.3,2.8984778792367));
#4124=CARTESIAN_POINT('',(0.480374109850668,-0.48,2.85950064615405));
#4125=CARTESIAN_POINT('Origin',(0.747146023568809,0.3,2.43463319293926));
#4126=CARTESIAN_POINT('',(1.26019081042021,0.3,1.98821965519135));
#4127=CARTESIAN_POINT('',(1.26019081042021,0.3,1.98821965519135));
#4128=CARTESIAN_POINT('',(0.410649515652541,0.3,2.06254488768065));
#4129=CARTESIAN_POINT('',(1.45942975003856,0.3,1.97078850664181));
#4130=CARTESIAN_POINT('Origin',(0.,0.3,2.5));
#4131=CARTESIAN_POINT('Origin',(1.45942975003856,-0.3,1.97078850664181));
#4132=CARTESIAN_POINT('',(1.26019081042021,-0.6,1.98821965519135));
#4133=CARTESIAN_POINT('',(0.410649515652541,-0.48,2.06254488768065));
#4134=CARTESIAN_POINT('Origin',(0.,-0.48,2.5));
#4135=CARTESIAN_POINT('',(-0.6,0.48,2.5));
#4136=CARTESIAN_POINT('Origin',(0.,0.48,2.5));
#4137=CARTESIAN_POINT('',(-0.6,-0.48,2.5));
#4138=CARTESIAN_POINT('',(-0.6,-0.48,2.5));
#4139=CARTESIAN_POINT('Origin',(0.,-0.48,2.5));
#4140=CARTESIAN_POINT('Origin',(0.,0.48,2.5));
#4141=CARTESIAN_POINT('Origin',(0.,-0.48,2.5));
#4142=CARTESIAN_POINT('Origin',(3.21771790950463,-0.9,1.41543029045933));
#4143=CARTESIAN_POINT('',(3.21771790950463,-0.5,1.41543029045933));
#4144=CARTESIAN_POINT('',(1.22532851332114,-0.5,1.58974177595465));
#4145=CARTESIAN_POINT('',(3.21771790950463,-0.9,1.41543029045933));
#4146=CARTESIAN_POINT('',(3.21771790950463,-0.9,1.41543029045933));
#4147=CARTESIAN_POINT('',(1.22532851332114,-0.9,1.58974177595465));
#4148=CARTESIAN_POINT('',(1.22532851332114,-0.9,1.58974177595465));
#4149=CARTESIAN_POINT('',(1.22532851332114,-0.9,1.58974177595465));
#4150=CARTESIAN_POINT('Origin',(2.29124780561101,-0.5,2.29954179168039));
#4151=CARTESIAN_POINT('',(3.35716709790089,-0.5,3.00934180740612));
#4152=CARTESIAN_POINT('',(3.35716709790089,-0.5,3.00934180740612));
#4153=CARTESIAN_POINT('',(3.21771790950463,-0.5,1.41543029045933));
#4154=CARTESIAN_POINT('Origin',(1.22532851332114,-0.9,1.58974177595465));
#4155=CARTESIAN_POINT('',(1.3647777017174,-0.9,3.18365329290144));
#4156=CARTESIAN_POINT('',(1.3647777017174,-0.9,3.18365329290144));
#4157=CARTESIAN_POINT('',(1.3647777017174,-0.9,3.18365329290144));
#4158=CARTESIAN_POINT('Origin',(3.35716709790089,-0.9,3.00934180740612));
#4159=CARTESIAN_POINT('',(3.35716709790089,-0.9,3.00934180740612));
#4160=CARTESIAN_POINT('',(3.21771790950463,-0.9,1.41543029045933));
#4161=CARTESIAN_POINT('',(3.35716709790089,-0.9,3.00934180740612));
#4162=CARTESIAN_POINT('Origin',(1.3647777017174,-0.9,3.18365329290144));
#4163=CARTESIAN_POINT('',(3.35716709790089,-0.9,3.00934180740612));
#4164=CARTESIAN_POINT('Origin',(2.29124780561101,-0.9,2.29954179168039));
#4758=UNCERTAINTY_MEASURE_WITH_UNIT(LENGTH_MEASURE(0.001),#4792,
'DISTANCE_ACCURACY_VALUE',
'Maximum model space distance between geometric entities at asserted c
onnectivities');
#4772=UNCERTAINTY_MEASURE_WITH_UNIT(LENGTH_MEASURE(0.001),#4792,
'DISTANCE_ACCURACY_VALUE',
'Maximum model space distance between geometric entities at asserted c
onnectivities');
#4777=(
GEOMETRIC_REPRESENTATION_CONTEXT(3)
GLOBAL_UNCERTAINTY_ASSIGNED_CONTEXT((#4758))
GLOBAL_UNIT_ASSIGNED_CONTEXT((#4792,#4794,#4795))
REPRESENTATION_CONTEXT('','3D')
);
#4791=(
GEOMETRIC_REPRESENTATION_CONTEXT(3)
GLOBAL_UNCERTAINTY_ASSIGNED_CONTEXT((#4772))
GLOBAL_UNIT_ASSIGNED_CONTEXT((#4792,#4794,#4795))
REPRESENTATION_CONTEXT('','3D')
);
#4792=(
LENGTH_UNIT()
NAMED_UNIT(*)
SI_UNIT(.CENTI.,.METRE.)
);
#4794=(
NAMED_UNIT(*)
PLANE_ANGLE_UNIT()
SI_UNIT($,.RADIAN.)
);
#4795=(
NAMED_UNIT(*)
SI_UNIT($,.STERADIAN.)
SOLID_ANGLE_UNIT()
);
#4800=SHAPE_DEFINITION_REPRESENTATION(#4818,#4864);
#4818=PRODUCT_DEFINITION_SHAPE('',$,#4883);
#4864=SHAPE_REPRESENTATION('',(#2838),#4777);
#4878=PRODUCT_DEFINITION_CONTEXT('part definition',#4934,'design');
#4883=PRODUCT_DEFINITION('Operating lever','Operating lever',#4901,#4878);
#4901=PRODUCT_DEFINITION_FORMATION('',$,#4940);
#4934=APPLICATION_CONTEXT(
'Core Data for Automotive Mechanical Design Process');
#4935=PRODUCT_CONTEXT('part definition',#4934,'mechanical');
#4940=PRODUCT('Operating lever','Operating lever','Operating lever',(#4935));
#5003=COLOUR_RGB('Light Blue',0.38,0.62,0.78);
#5004=FILL_AREA_STYLE_COLOUR('',#5003);
#5005=FILL_AREA_STYLE('',(#5004));
#5006=SURFACE_STYLE_FILL_AREA(#5005);
#5007=SURFACE_SIDE_STYLE('',(#5006));
#5008=SURFACE_STYLE_USAGE(.BOTH.,#5007);
#5009=PRESENTATION_STYLE_ASSIGNMENT((#5008));
ENDSEC;
END-ISO-10303-21;
